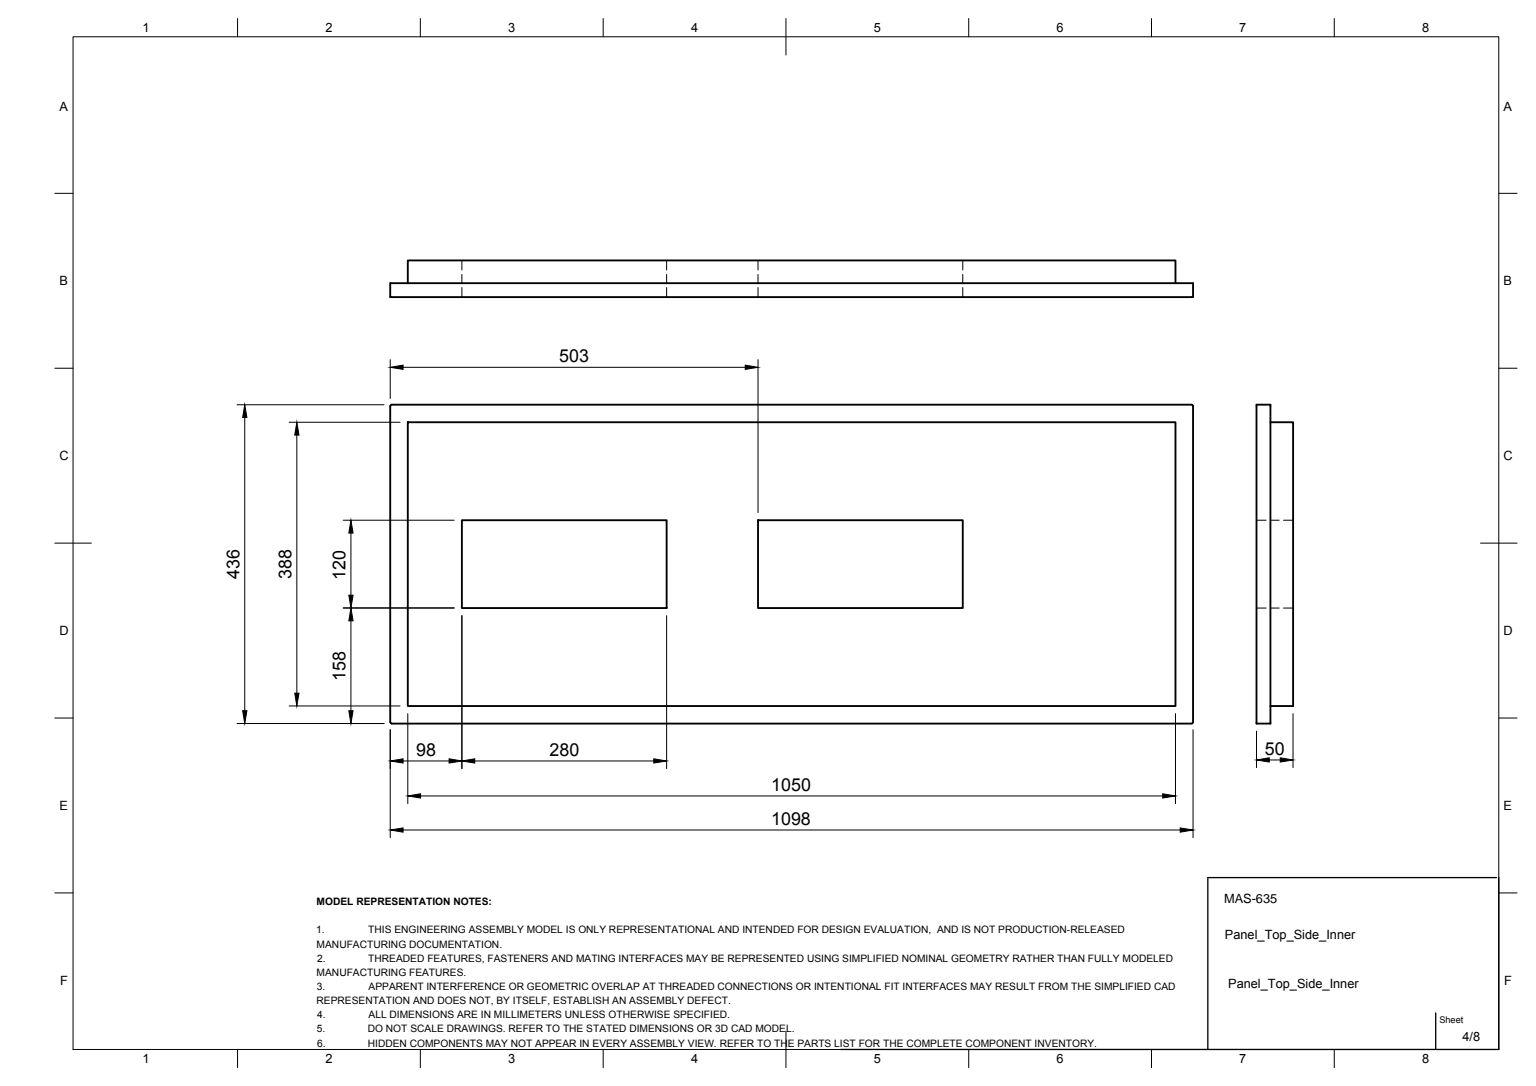
ISO-10303-21;
HEADER;
FILE_DESCRIPTION((''),'2;1');
FILE_NAME('Panel_Top_Side_Inner.step','2026-10-09T12:34:24-07:00',(''),(''),'','','');
FILE_SCHEMA (('AUTOMOTIVE_DESIGN { 1 0 10303 214 3 1 1 }'));
ENDSEC;
DATA;
#10=MECHANICAL_DESIGN_GEOMETRIC_PRESENTATION_REPRESENTATION('',(#60),#3759);
#48=SHAPE_REPRESENTATION_RELATIONSHIP('SRR','None',#3789,#54) ;
#54=ADVANCED_BREP_SHAPE_REPRESENTATION('',(#66),#3754) ;
#60=STYLED_ITEM('',(#3827),#66) ;
#66=MANIFOLD_SOLID_BREP('Body1',#2264) ;
#75=CYLINDRICAL_SURFACE('',#2389,0.2) ;
#76=CYLINDRICAL_SURFACE('',#2390,0.2) ;
#77=CYLINDRICAL_SURFACE('',#2391,0.2) ;
#78=CYLINDRICAL_SURFACE('',#2392,0.2) ;
#95=CIRCLE('',#2380,0.2) ;
#96=CIRCLE('',#2381,0.2) ;
#97=CIRCLE('',#2382,0.2) ;
#98=CIRCLE('',#2383,0.2) ;
#99=CIRCLE('',#2385,0.2) ;
#100=CIRCLE('',#2386,0.2) ;
#101=CIRCLE('',#2387,0.2) ;
#102=CIRCLE('',#2388,0.2) ;
#124=FACE_BOUND('',#294,.T.) ;
#125=FACE_BOUND('',#295,.T.) ;
#126=FACE_BOUND('',#301,.T.) ;
#127=FACE_BOUND('',#303,.T.) ;
#128=FACE_BOUND('',#304,.T.) ;
#164=FACE_OUTER_BOUND('',#289,.T.) ;
#165=FACE_OUTER_BOUND('',#290,.T.) ;
#166=FACE_OUTER_BOUND('',#291,.T.) ;
#167=FACE_OUTER_BOUND('',#292,.T.) ;
#168=FACE_OUTER_BOUND('',#293,.T.) ;
#169=FACE_OUTER_BOUND('',#296,.T.) ;
#170=FACE_OUTER_BOUND('',#297,.T.) ;
#171=FACE_OUTER_BOUND('',#298,.T.) ;
#172=FACE_OUTER_BOUND('',#299,.T.) ;
#173=FACE_OUTER_BOUND('',#300,.T.) ;
#174=FACE_OUTER_BOUND('',#302,.T.) ;
#175=FACE_OUTER_BOUND('',#305,.T.) ;
#176=FACE_OUTER_BOUND('',#306,.T.) ;
#177=FACE_OUTER_BOUND('',#307,.T.) ;
#178=FACE_OUTER_BOUND('',#308,.T.) ;
#179=FACE_OUTER_BOUND('',#309,.T.) ;
#180=FACE_OUTER_BOUND('',#310,.T.) ;
#181=FACE_OUTER_BOUND('',#311,.T.) ;
#182=FACE_OUTER_BOUND('',#312,.T.) ;
#183=FACE_OUTER_BOUND('',#313,.T.) ;
#184=FACE_OUTER_BOUND('',#314,.T.) ;
#185=FACE_OUTER_BOUND('',#315,.T.) ;
#186=FACE_OUTER_BOUND('',#316,.T.) ;
#289=EDGE_LOOP('',(#1559,#1560,#1561,#1562)) ;
#290=EDGE_LOOP('',(#1563,#1564,#1565,#1566)) ;
#291=EDGE_LOOP('',(#1567,#1568,#1569,#1570)) ;
#292=EDGE_LOOP('',(#1571,#1572,#1573,#1574)) ;
#293=EDGE_LOOP('',(#1575,#1576,#1577,#1578)) ;
#294=EDGE_LOOP('',(#1579,#1580,#1581,#1582)) ;
#295=EDGE_LOOP('',(#1583,#1584,#1585,#1586)) ;
#296=EDGE_LOOP('',(#1587,#1588,#1589,#1590)) ;
#297=EDGE_LOOP('',(#1591,#1592,#1593,#1594)) ;
#298=EDGE_LOOP('',(#1595,#1596,#1597,#1598)) ;
#299=EDGE_LOOP('',(#1599,#1600,#1601,#1602)) ;
#300=EDGE_LOOP('',(#1603,#1604,#1605,#1606,#1607,#1608,#1609,#1610)) ;
#301=EDGE_LOOP('',(#1611,#1612,#1613,#1614)) ;
#302=EDGE_LOOP('',(#1615,#1616,#1617,#1618,#1619,#1620,#1621,#1622)) ;
#303=EDGE_LOOP('',(#1623,#1624,#1625,#1626)) ;
#304=EDGE_LOOP('',(#1627,#1628,#1629,#1630)) ;
#305=EDGE_LOOP('',(#1631,#1632,#1633,#1634)) ;
#306=EDGE_LOOP('',(#1635,#1636,#1637,#1638)) ;
#307=EDGE_LOOP('',(#1639,#1640,#1641,#1642)) ;
#308=EDGE_LOOP('',(#1643,#1644,#1645,#1646)) ;
#309=EDGE_LOOP('',(#1647,#1648,#1649,#1650)) ;
#310=EDGE_LOOP('',(#1651,#1652,#1653,#1654)) ;
#311=EDGE_LOOP('',(#1655,#1656,#1657,#1658)) ;
#312=EDGE_LOOP('',(#1659,#1660,#1661,#1662)) ;
#313=EDGE_LOOP('',(#1663,#1664,#1665,#1666)) ;
#314=EDGE_LOOP('',(#1667,#1668,#1669,#1670)) ;
#315=EDGE_LOOP('',(#1671,#1672,#1673,#1674)) ;
#316=EDGE_LOOP('',(#1675,#1676,#1677,#1678)) ;
#455=LINE('',#3237,#723) ;
#456=LINE('',#3239,#724) ;
#457=LINE('',#3241,#725) ;
#458=LINE('',#3242,#726) ;
#459=LINE('',#3245,#727) ;
#460=LINE('',#3247,#728) ;
#461=LINE('',#3248,#729) ;
#462=LINE('',#3251,#730) ;
#463=LINE('',#3253,#731) ;
#464=LINE('',#3254,#732) ;
#465=LINE('',#3256,#733) ;
#466=LINE('',#3257,#734) ;
#467=LINE('',#3261,#735) ;
#468=LINE('',#3263,#736) ;
#469=LINE('',#3265,#737) ;
#470=LINE('',#3266,#738) ;
#471=LINE('',#3269,#739) ;
#472=LINE('',#3271,#740) ;
#473=LINE('',#3273,#741) ;
#474=LINE('',#3274,#742) ;
#475=LINE('',#3278,#743) ;
#476=LINE('',#3280,#744) ;
#477=LINE('',#3282,#745) ;
#478=LINE('',#3283,#746) ;
#479=LINE('',#3287,#747) ;
#480=LINE('',#3289,#748) ;
#481=LINE('',#3291,#749) ;
#482=LINE('',#3292,#750) ;
#483=LINE('',#3296,#751) ;
#484=LINE('',#3298,#752) ;
#485=LINE('',#3300,#753) ;
#486=LINE('',#3301,#754) ;
#487=LINE('',#3305,#755) ;
#488=LINE('',#3307,#756) ;
#489=LINE('',#3309,#757) ;
#490=LINE('',#3310,#758) ;
#491=LINE('',#3323,#759) ;
#492=LINE('',#3325,#760) ;
#493=LINE('',#3327,#761) ;
#494=LINE('',#3328,#762) ;
#495=LINE('',#3331,#763) ;
#496=LINE('',#3333,#764) ;
#497=LINE('',#3335,#765) ;
#498=LINE('',#3336,#766) ;
#499=LINE('',#3342,#767) ;
#500=LINE('',#3343,#768) ;
#501=LINE('',#3345,#769) ;
#502=LINE('',#3347,#770) ;
#503=LINE('',#3350,#771) ;
#504=LINE('',#3351,#772) ;
#505=LINE('',#3353,#773) ;
#506=LINE('',#3355,#774) ;
#723=VECTOR('',#2626,100.) ;
#724=VECTOR('',#2627,100.) ;
#725=VECTOR('',#2628,100.) ;
#726=VECTOR('',#2629,100.) ;
#727=VECTOR('',#2632,100.) ;
#728=VECTOR('',#2633,100.) ;
#729=VECTOR('',#2634,100.) ;
#730=VECTOR('',#2637,100.) ;
#731=VECTOR('',#2638,100.) ;
#732=VECTOR('',#2639,100.) ;
#733=VECTOR('',#2642,100.) ;
#734=VECTOR('',#2643,100.) ;
#735=VECTOR('',#2646,100.) ;
#736=VECTOR('',#2647,100.) ;
#737=VECTOR('',#2648,100.) ;
#738=VECTOR('',#2649,100.) ;
#739=VECTOR('',#2650,100.) ;
#740=VECTOR('',#2651,100.) ;
#741=VECTOR('',#2652,100.) ;
#742=VECTOR('',#2653,100.) ;
#743=VECTOR('',#2656,100.) ;
#744=VECTOR('',#2657,100.) ;
#745=VECTOR('',#2658,100.) ;
#746=VECTOR('',#2659,100.) ;
#747=VECTOR('',#2662,100.) ;
#748=VECTOR('',#2663,100.) ;
#749=VECTOR('',#2664,100.) ;
#750=VECTOR('',#2665,100.) ;
#751=VECTOR('',#2668,100.) ;
#752=VECTOR('',#2669,100.) ;
#753=VECTOR('',#2670,100.) ;
#754=VECTOR('',#2671,100.) ;
#755=VECTOR('',#2674,100.) ;
#756=VECTOR('',#2675,100.) ;
#757=VECTOR('',#2676,100.) ;
#758=VECTOR('',#2677,100.) ;
#759=VECTOR('',#2698,100.) ;
#760=VECTOR('',#2699,100.) ;
#761=VECTOR('',#2700,100.) ;
#762=VECTOR('',#2701,100.) ;
#763=VECTOR('',#2702,100.) ;
#764=VECTOR('',#2703,100.) ;
#765=VECTOR('',#2704,100.) ;
#766=VECTOR('',#2705,100.) ;
#767=VECTOR('',#2716,100.) ;
#768=VECTOR('',#2717,100.) ;
#769=VECTOR('',#2720,100.) ;
#770=VECTOR('',#2723,100.) ;
#771=VECTOR('',#2728,100.) ;
#772=VECTOR('',#2729,100.) ;
#773=VECTOR('',#2732,100.) ;
#774=VECTOR('',#2735,100.) ;
#979=VERTEX_POINT('',#3235) ;
#980=VERTEX_POINT('',#3236) ;
#981=VERTEX_POINT('',#3238) ;
#982=VERTEX_POINT('',#3240) ;
#983=VERTEX_POINT('',#3244) ;
#984=VERTEX_POINT('',#3246) ;
#985=VERTEX_POINT('',#3250) ;
#986=VERTEX_POINT('',#3252) ;
#987=VERTEX_POINT('',#3259) ;
#988=VERTEX_POINT('',#3260) ;
#989=VERTEX_POINT('',#3262) ;
#990=VERTEX_POINT('',#3264) ;
#991=VERTEX_POINT('',#3267) ;
#992=VERTEX_POINT('',#3268) ;
#993=VERTEX_POINT('',#3270) ;
#994=VERTEX_POINT('',#3272) ;
#995=VERTEX_POINT('',#3276) ;
#996=VERTEX_POINT('',#3277) ;
#997=VERTEX_POINT('',#3279) ;
#998=VERTEX_POINT('',#3281) ;
#999=VERTEX_POINT('',#3285) ;
#1000=VERTEX_POINT('',#3286) ;
#1001=VERTEX_POINT('',#3288) ;
#1002=VERTEX_POINT('',#3290) ;
#1003=VERTEX_POINT('',#3294) ;
#1004=VERTEX_POINT('',#3295) ;
#1005=VERTEX_POINT('',#3297) ;
#1006=VERTEX_POINT('',#3299) ;
#1007=VERTEX_POINT('',#3303) ;
#1008=VERTEX_POINT('',#3304) ;
#1009=VERTEX_POINT('',#3306) ;
#1010=VERTEX_POINT('',#3308) ;
#1011=VERTEX_POINT('',#3321) ;
#1012=VERTEX_POINT('',#3322) ;
#1013=VERTEX_POINT('',#3324) ;
#1014=VERTEX_POINT('',#3326) ;
#1015=VERTEX_POINT('',#3329) ;
#1016=VERTEX_POINT('',#3330) ;
#1017=VERTEX_POINT('',#3332) ;
#1018=VERTEX_POINT('',#3334) ;
#1199=EDGE_CURVE('',#979,#980,#455,.T.) ;
#1200=EDGE_CURVE('',#981,#979,#456,.T.) ;
#1201=EDGE_CURVE('',#981,#982,#457,.T.) ;
#1202=EDGE_CURVE('',#982,#980,#458,.T.) ;
#1203=EDGE_CURVE('',#979,#983,#459,.T.) ;
#1204=EDGE_CURVE('',#984,#983,#460,.T.) ;
#1205=EDGE_CURVE('',#981,#984,#461,.T.) ;
#1206=EDGE_CURVE('',#983,#985,#462,.T.) ;
#1207=EDGE_CURVE('',#986,#985,#463,.T.) ;
#1208=EDGE_CURVE('',#984,#986,#464,.T.) ;
#1209=EDGE_CURVE('',#980,#985,#465,.T.) ;
#1210=EDGE_CURVE('',#982,#986,#466,.T.) ;
#1211=EDGE_CURVE('',#987,#988,#467,.T.) ;
#1212=EDGE_CURVE('',#988,#989,#468,.T.) ;
#1213=EDGE_CURVE('',#989,#990,#469,.T.) ;
#1214=EDGE_CURVE('',#990,#987,#470,.T.) ;
#1215=EDGE_CURVE('',#991,#992,#471,.T.) ;
#1216=EDGE_CURVE('',#992,#993,#472,.T.) ;
#1217=EDGE_CURVE('',#993,#994,#473,.T.) ;
#1218=EDGE_CURVE('',#994,#991,#474,.T.) ;
#1219=EDGE_CURVE('',#995,#996,#475,.T.) ;
#1220=EDGE_CURVE('',#995,#997,#476,.T.) ;
#1221=EDGE_CURVE('',#997,#998,#477,.T.) ;
#1222=EDGE_CURVE('',#998,#996,#478,.T.) ;
#1223=EDGE_CURVE('',#999,#1000,#479,.T.) ;
#1224=EDGE_CURVE('',#1000,#1001,#480,.T.) ;
#1225=EDGE_CURVE('',#1002,#1001,#481,.T.) ;
#1226=EDGE_CURVE('',#1002,#999,#482,.T.) ;
#1227=EDGE_CURVE('',#1003,#1004,#483,.T.) ;
#1228=EDGE_CURVE('',#1003,#1005,#484,.T.) ;
#1229=EDGE_CURVE('',#1005,#1006,#485,.T.) ;
#1230=EDGE_CURVE('',#1006,#1004,#486,.T.) ;
#1231=EDGE_CURVE('',#1007,#1008,#487,.T.) ;
#1232=EDGE_CURVE('',#1007,#1009,#488,.T.) ;
#1233=EDGE_CURVE('',#1009,#1010,#489,.T.) ;
#1234=EDGE_CURVE('',#1010,#1008,#490,.T.) ;
#1235=EDGE_CURVE('',#1009,#995,#95,.T.) ;
#1236=EDGE_CURVE('',#996,#1002,#96,.T.) ;
#1237=EDGE_CURVE('',#1001,#1006,#97,.T.) ;
#1238=EDGE_CURVE('',#1005,#1010,#98,.T.) ;
#1239=EDGE_CURVE('',#997,#1007,#99,.T.) ;
#1240=EDGE_CURVE('',#1008,#1003,#100,.T.) ;
#1241=EDGE_CURVE('',#1004,#1000,#101,.T.) ;
#1242=EDGE_CURVE('',#999,#998,#102,.T.) ;
#1243=EDGE_CURVE('',#1011,#1012,#491,.T.) ;
#1244=EDGE_CURVE('',#1013,#1011,#492,.T.) ;
#1245=EDGE_CURVE('',#1014,#1013,#493,.T.) ;
#1246=EDGE_CURVE('',#1012,#1014,#494,.T.) ;
#1247=EDGE_CURVE('',#1015,#1016,#495,.T.) ;
#1248=EDGE_CURVE('',#1017,#1015,#496,.T.) ;
#1249=EDGE_CURVE('',#1018,#1017,#497,.T.) ;
#1250=EDGE_CURVE('',#1016,#1018,#498,.T.) ;
#1251=EDGE_CURVE('',#992,#1015,#499,.T.) ;
#1252=EDGE_CURVE('',#993,#1016,#500,.T.) ;
#1253=EDGE_CURVE('',#991,#1017,#501,.T.) ;
#1254=EDGE_CURVE('',#994,#1018,#502,.T.) ;
#1255=EDGE_CURVE('',#988,#1011,#503,.T.) ;
#1256=EDGE_CURVE('',#989,#1012,#504,.T.) ;
#1257=EDGE_CURVE('',#987,#1013,#505,.T.) ;
#1258=EDGE_CURVE('',#990,#1014,#506,.T.) ;
#1559=ORIENTED_EDGE('',*,*,#1199,.F.) ;
#1560=ORIENTED_EDGE('',*,*,#1200,.F.) ;
#1561=ORIENTED_EDGE('',*,*,#1201,.T.) ;
#1562=ORIENTED_EDGE('',*,*,#1202,.T.) ;
#1563=ORIENTED_EDGE('',*,*,#1200,.T.) ;
#1564=ORIENTED_EDGE('',*,*,#1203,.T.) ;
#1565=ORIENTED_EDGE('',*,*,#1204,.F.) ;
#1566=ORIENTED_EDGE('',*,*,#1205,.F.) ;
#1567=ORIENTED_EDGE('',*,*,#1204,.T.) ;
#1568=ORIENTED_EDGE('',*,*,#1206,.T.) ;
#1569=ORIENTED_EDGE('',*,*,#1207,.F.) ;
#1570=ORIENTED_EDGE('',*,*,#1208,.F.) ;
#1571=ORIENTED_EDGE('',*,*,#1209,.F.) ;
#1572=ORIENTED_EDGE('',*,*,#1202,.F.) ;
#1573=ORIENTED_EDGE('',*,*,#1210,.T.) ;
#1574=ORIENTED_EDGE('',*,*,#1207,.T.) ;
#1575=ORIENTED_EDGE('',*,*,#1201,.F.) ;
#1576=ORIENTED_EDGE('',*,*,#1205,.T.) ;
#1577=ORIENTED_EDGE('',*,*,#1208,.T.) ;
#1578=ORIENTED_EDGE('',*,*,#1210,.F.) ;
#1579=ORIENTED_EDGE('',*,*,#1211,.T.) ;
#1580=ORIENTED_EDGE('',*,*,#1212,.T.) ;
#1581=ORIENTED_EDGE('',*,*,#1213,.T.) ;
#1582=ORIENTED_EDGE('',*,*,#1214,.T.) ;
#1583=ORIENTED_EDGE('',*,*,#1215,.T.) ;
#1584=ORIENTED_EDGE('',*,*,#1216,.T.) ;
#1585=ORIENTED_EDGE('',*,*,#1217,.T.) ;
#1586=ORIENTED_EDGE('',*,*,#1218,.T.) ;
#1587=ORIENTED_EDGE('',*,*,#1219,.F.) ;
#1588=ORIENTED_EDGE('',*,*,#1220,.T.) ;
#1589=ORIENTED_EDGE('',*,*,#1221,.T.) ;
#1590=ORIENTED_EDGE('',*,*,#1222,.T.) ;
#1591=ORIENTED_EDGE('',*,*,#1223,.T.) ;
#1592=ORIENTED_EDGE('',*,*,#1224,.T.) ;
#1593=ORIENTED_EDGE('',*,*,#1225,.F.) ;
#1594=ORIENTED_EDGE('',*,*,#1226,.T.) ;
#1595=ORIENTED_EDGE('',*,*,#1227,.F.) ;
#1596=ORIENTED_EDGE('',*,*,#1228,.T.) ;
#1597=ORIENTED_EDGE('',*,*,#1229,.T.) ;
#1598=ORIENTED_EDGE('',*,*,#1230,.T.) ;
#1599=ORIENTED_EDGE('',*,*,#1231,.F.) ;
#1600=ORIENTED_EDGE('',*,*,#1232,.T.) ;
#1601=ORIENTED_EDGE('',*,*,#1233,.T.) ;
#1602=ORIENTED_EDGE('',*,*,#1234,.T.) ;
#1603=ORIENTED_EDGE('',*,*,#1233,.F.) ;
#1604=ORIENTED_EDGE('',*,*,#1235,.T.) ;
#1605=ORIENTED_EDGE('',*,*,#1219,.T.) ;
#1606=ORIENTED_EDGE('',*,*,#1236,.T.) ;
#1607=ORIENTED_EDGE('',*,*,#1225,.T.) ;
#1608=ORIENTED_EDGE('',*,*,#1237,.T.) ;
#1609=ORIENTED_EDGE('',*,*,#1229,.F.) ;
#1610=ORIENTED_EDGE('',*,*,#1238,.T.) ;
#1611=ORIENTED_EDGE('',*,*,#1203,.F.) ;
#1612=ORIENTED_EDGE('',*,*,#1199,.T.) ;
#1613=ORIENTED_EDGE('',*,*,#1209,.T.) ;
#1614=ORIENTED_EDGE('',*,*,#1206,.F.) ;
#1615=ORIENTED_EDGE('',*,*,#1221,.F.) ;
#1616=ORIENTED_EDGE('',*,*,#1239,.T.) ;
#1617=ORIENTED_EDGE('',*,*,#1231,.T.) ;
#1618=ORIENTED_EDGE('',*,*,#1240,.T.) ;
#1619=ORIENTED_EDGE('',*,*,#1227,.T.) ;
#1620=ORIENTED_EDGE('',*,*,#1241,.T.) ;
#1621=ORIENTED_EDGE('',*,*,#1223,.F.) ;
#1622=ORIENTED_EDGE('',*,*,#1242,.T.) ;
#1623=ORIENTED_EDGE('',*,*,#1243,.F.) ;
#1624=ORIENTED_EDGE('',*,*,#1244,.F.) ;
#1625=ORIENTED_EDGE('',*,*,#1245,.F.) ;
#1626=ORIENTED_EDGE('',*,*,#1246,.F.) ;
#1627=ORIENTED_EDGE('',*,*,#1247,.F.) ;
#1628=ORIENTED_EDGE('',*,*,#1248,.F.) ;
#1629=ORIENTED_EDGE('',*,*,#1249,.F.) ;
#1630=ORIENTED_EDGE('',*,*,#1250,.F.) ;
#1631=ORIENTED_EDGE('',*,*,#1235,.F.) ;
#1632=ORIENTED_EDGE('',*,*,#1232,.F.) ;
#1633=ORIENTED_EDGE('',*,*,#1239,.F.) ;
#1634=ORIENTED_EDGE('',*,*,#1220,.F.) ;
#1635=ORIENTED_EDGE('',*,*,#1238,.F.) ;
#1636=ORIENTED_EDGE('',*,*,#1228,.F.) ;
#1637=ORIENTED_EDGE('',*,*,#1240,.F.) ;
#1638=ORIENTED_EDGE('',*,*,#1234,.F.) ;
#1639=ORIENTED_EDGE('',*,*,#1237,.F.) ;
#1640=ORIENTED_EDGE('',*,*,#1224,.F.) ;
#1641=ORIENTED_EDGE('',*,*,#1241,.F.) ;
#1642=ORIENTED_EDGE('',*,*,#1230,.F.) ;
#1643=ORIENTED_EDGE('',*,*,#1236,.F.) ;
#1644=ORIENTED_EDGE('',*,*,#1222,.F.) ;
#1645=ORIENTED_EDGE('',*,*,#1242,.F.) ;
#1646=ORIENTED_EDGE('',*,*,#1226,.F.) ;
#1647=ORIENTED_EDGE('',*,*,#1251,.T.) ;
#1648=ORIENTED_EDGE('',*,*,#1247,.T.) ;
#1649=ORIENTED_EDGE('',*,*,#1252,.F.) ;
#1650=ORIENTED_EDGE('',*,*,#1216,.F.) ;
#1651=ORIENTED_EDGE('',*,*,#1253,.T.) ;
#1652=ORIENTED_EDGE('',*,*,#1248,.T.) ;
#1653=ORIENTED_EDGE('',*,*,#1251,.F.) ;
#1654=ORIENTED_EDGE('',*,*,#1215,.F.) ;
#1655=ORIENTED_EDGE('',*,*,#1254,.T.) ;
#1656=ORIENTED_EDGE('',*,*,#1249,.T.) ;
#1657=ORIENTED_EDGE('',*,*,#1253,.F.) ;
#1658=ORIENTED_EDGE('',*,*,#1218,.F.) ;
#1659=ORIENTED_EDGE('',*,*,#1252,.T.) ;
#1660=ORIENTED_EDGE('',*,*,#1250,.T.) ;
#1661=ORIENTED_EDGE('',*,*,#1254,.F.) ;
#1662=ORIENTED_EDGE('',*,*,#1217,.F.) ;
#1663=ORIENTED_EDGE('',*,*,#1255,.T.) ;
#1664=ORIENTED_EDGE('',*,*,#1243,.T.) ;
#1665=ORIENTED_EDGE('',*,*,#1256,.F.) ;
#1666=ORIENTED_EDGE('',*,*,#1212,.F.) ;
#1667=ORIENTED_EDGE('',*,*,#1257,.T.) ;
#1668=ORIENTED_EDGE('',*,*,#1244,.T.) ;
#1669=ORIENTED_EDGE('',*,*,#1255,.F.) ;
#1670=ORIENTED_EDGE('',*,*,#1211,.F.) ;
#1671=ORIENTED_EDGE('',*,*,#1258,.T.) ;
#1672=ORIENTED_EDGE('',*,*,#1245,.T.) ;
#1673=ORIENTED_EDGE('',*,*,#1257,.F.) ;
#1674=ORIENTED_EDGE('',*,*,#1214,.F.) ;
#1675=ORIENTED_EDGE('',*,*,#1256,.T.) ;
#1676=ORIENTED_EDGE('',*,*,#1246,.T.) ;
#1677=ORIENTED_EDGE('',*,*,#1258,.F.) ;
#1678=ORIENTED_EDGE('',*,*,#1213,.F.) ;
#2058=PLANE('',#2370) ;
#2059=PLANE('',#2371) ;
#2060=PLANE('',#2372) ;
#2061=PLANE('',#2373) ;
#2062=PLANE('',#2374) ;
#2063=PLANE('',#2375) ;
#2064=PLANE('',#2376) ;
#2065=PLANE('',#2377) ;
#2066=PLANE('',#2378) ;
#2067=PLANE('',#2379) ;
#2068=PLANE('',#2384) ;
#2069=PLANE('',#2393) ;
#2070=PLANE('',#2394) ;
#2071=PLANE('',#2395) ;
#2072=PLANE('',#2396) ;
#2073=PLANE('',#2397) ;
#2074=PLANE('',#2398) ;
#2075=PLANE('',#2399) ;
#2076=PLANE('',#2400) ;
#2166=ADVANCED_FACE('',(#164),#2058,.T.) ;
#2167=ADVANCED_FACE('',(#165),#2059,.F.) ;
#2168=ADVANCED_FACE('',(#166),#2060,.F.) ;
#2169=ADVANCED_FACE('',(#167),#2061,.T.) ;
#2170=ADVANCED_FACE('',(#168,#124,#125),#2062,.F.) ;
#2171=ADVANCED_FACE('',(#169),#2063,.F.) ;
#2172=ADVANCED_FACE('',(#170),#2064,.F.) ;
#2173=ADVANCED_FACE('',(#171),#2065,.T.) ;
#2174=ADVANCED_FACE('',(#172),#2066,.T.) ;
#2175=ADVANCED_FACE('',(#173,#126),#2067,.T.) ;
#2176=ADVANCED_FACE('',(#174,#127,#128),#2068,.T.) ;
#2177=ADVANCED_FACE('',(#175),#75,.T.) ;
#2178=ADVANCED_FACE('',(#176),#76,.T.) ;
#2179=ADVANCED_FACE('',(#177),#77,.T.) ;
#2180=ADVANCED_FACE('',(#178),#78,.T.) ;
#2181=ADVANCED_FACE('',(#179),#2069,.F.) ;
#2182=ADVANCED_FACE('',(#180),#2070,.F.) ;
#2183=ADVANCED_FACE('',(#181),#2071,.F.) ;
#2184=ADVANCED_FACE('',(#182),#2072,.F.) ;
#2185=ADVANCED_FACE('',(#183),#2073,.F.) ;
#2186=ADVANCED_FACE('',(#184),#2074,.F.) ;
#2187=ADVANCED_FACE('',(#185),#2075,.F.) ;
#2188=ADVANCED_FACE('',(#186),#2076,.F.) ;
#2264=CLOSED_SHELL('',(#2166,#2167,#2168,#2169,#2170,#2171,#2172,#2173,
#2174,#2175,#2176,#2177,#2178,#2179,#2180,#2181,#2182,#2183,#2184,#2185,
#2186,#2187,#2188)) ;
#2369=AXIS2_PLACEMENT_3D('',#3233,#2622,#2623) ;
#2370=AXIS2_PLACEMENT_3D('',#3234,#2624,#2625) ;
#2371=AXIS2_PLACEMENT_3D('',#3243,#2630,#2631) ;
#2372=AXIS2_PLACEMENT_3D('',#3249,#2635,#2636) ;
#2373=AXIS2_PLACEMENT_3D('',#3255,#2640,#2641) ;
#2374=AXIS2_PLACEMENT_3D('',#3258,#2644,#2645) ;
#2375=AXIS2_PLACEMENT_3D('',#3275,#2654,#2655) ;
#2376=AXIS2_PLACEMENT_3D('',#3284,#2660,#2661) ;
#2377=AXIS2_PLACEMENT_3D('',#3293,#2666,#2667) ;
#2378=AXIS2_PLACEMENT_3D('',#3302,#2672,#2673) ;
#2379=AXIS2_PLACEMENT_3D('',#3311,#2678,#2679) ;
#2380=AXIS2_PLACEMENT_3D('',#3312,#2680,#2681) ;
#2381=AXIS2_PLACEMENT_3D('',#3313,#2682,#2683) ;
#2382=AXIS2_PLACEMENT_3D('',#3314,#2684,#2685) ;
#2383=AXIS2_PLACEMENT_3D('',#3315,#2686,#2687) ;
#2384=AXIS2_PLACEMENT_3D('',#3316,#2688,#2689) ;
#2385=AXIS2_PLACEMENT_3D('',#3317,#2690,#2691) ;
#2386=AXIS2_PLACEMENT_3D('',#3318,#2692,#2693) ;
#2387=AXIS2_PLACEMENT_3D('',#3319,#2694,#2695) ;
#2388=AXIS2_PLACEMENT_3D('',#3320,#2696,#2697) ;
#2389=AXIS2_PLACEMENT_3D('',#3337,#2706,#2707) ;
#2390=AXIS2_PLACEMENT_3D('',#3338,#2708,#2709) ;
#2391=AXIS2_PLACEMENT_3D('',#3339,#2710,#2711) ;
#2392=AXIS2_PLACEMENT_3D('',#3340,#2712,#2713) ;
#2393=AXIS2_PLACEMENT_3D('',#3341,#2714,#2715) ;
#2394=AXIS2_PLACEMENT_3D('',#3344,#2718,#2719) ;
#2395=AXIS2_PLACEMENT_3D('',#3346,#2721,#2722) ;
#2396=AXIS2_PLACEMENT_3D('',#3348,#2724,#2725) ;
#2397=AXIS2_PLACEMENT_3D('',#3349,#2726,#2727) ;
#2398=AXIS2_PLACEMENT_3D('',#3352,#2730,#2731) ;
#2399=AXIS2_PLACEMENT_3D('',#3354,#2733,#2734) ;
#2400=AXIS2_PLACEMENT_3D('',#3356,#2736,#2737) ;
#2622=DIRECTION('axis',(0.,0.,1.)) ;
#2623=DIRECTION('refdir',(1.,0.,0.)) ;
#2624=DIRECTION('center_axis',(1.58603289232165E-16,-1.,0.)) ;
#2625=DIRECTION('ref_axis',(1.,1.58603289232165E-16,0.)) ;
#2626=DIRECTION('',(-1.,-1.58603289232165E-16,0.)) ;
#2627=DIRECTION('',(0.,0.,-1.)) ;
#2628=DIRECTION('',(-1.,-1.58603289232165E-16,0.)) ;
#2629=DIRECTION('',(0.,0.,-1.)) ;
#2630=DIRECTION('center_axis',(-1.,0.,0.)) ;
#2631=DIRECTION('ref_axis',(0.,0.,1.)) ;
#2632=DIRECTION('',(0.,1.,0.)) ;
#2633=DIRECTION('',(0.,0.,-1.)) ;
#2634=DIRECTION('',(0.,1.,0.)) ;
#2635=DIRECTION('center_axis',(1.05735526154777E-16,-1.,0.)) ;
#2636=DIRECTION('ref_axis',(1.,1.05735526154777E-16,0.)) ;
#2637=DIRECTION('',(-1.,-1.05735526154777E-16,0.)) ;
#2638=DIRECTION('',(0.,0.,-1.)) ;
#2639=DIRECTION('',(-1.,-1.05735526154777E-16,0.)) ;
#2640=DIRECTION('center_axis',(-1.,0.,0.)) ;
#2641=DIRECTION('ref_axis',(0.,0.,1.)) ;
#2642=DIRECTION('',(0.,1.,0.)) ;
#2643=DIRECTION('',(0.,1.,0.)) ;
#2644=DIRECTION('center_axis',(0.,0.,-1.)) ;
#2645=DIRECTION('ref_axis',(-1.,0.,0.)) ;
#2646=DIRECTION('',(1.,-1.23908819712629E-16,0.)) ;
#2647=DIRECTION('',(0.,-1.,0.)) ;
#2648=DIRECTION('',(-1.,1.23908819712629E-16,0.)) ;
#2649=DIRECTION('',(0.,1.,0.)) ;
#2650=DIRECTION('',(-1.,0.,0.)) ;
#2651=DIRECTION('',(0.,1.,0.)) ;
#2652=DIRECTION('',(1.,0.,0.)) ;
#2653=DIRECTION('',(0.,-1.,0.)) ;
#2654=DIRECTION('center_axis',(-1.,0.,0.)) ;
#2655=DIRECTION('ref_axis',(0.,0.,1.)) ;
#2656=DIRECTION('',(0.,1.,0.)) ;
#2657=DIRECTION('',(0.,0.,-1.)) ;
#2658=DIRECTION('',(0.,1.,0.)) ;
#2659=DIRECTION('',(0.,0.,1.)) ;
#2660=DIRECTION('center_axis',(1.26391510089385E-16,-1.,0.)) ;
#2661=DIRECTION('ref_axis',(1.,1.26391510089385E-16,0.)) ;
#2662=DIRECTION('',(-1.,-1.26391510089385E-16,0.)) ;
#2663=DIRECTION('',(0.,0.,1.)) ;
#2664=DIRECTION('',(-1.,-1.26391510089385E-16,0.)) ;
#2665=DIRECTION('',(0.,0.,-1.)) ;
#2666=DIRECTION('center_axis',(-1.,0.,0.)) ;
#2667=DIRECTION('ref_axis',(0.,0.,1.)) ;
#2668=DIRECTION('',(0.,1.,0.)) ;
#2669=DIRECTION('',(0.,0.,1.)) ;
#2670=DIRECTION('',(0.,1.,0.)) ;
#2671=DIRECTION('',(0.,0.,-1.)) ;
#2672=DIRECTION('center_axis',(1.51669812107262E-16,-1.,0.)) ;
#2673=DIRECTION('ref_axis',(1.,1.51669812107262E-16,0.)) ;
#2674=DIRECTION('',(-1.,-1.51669812107262E-16,0.)) ;
#2675=DIRECTION('',(0.,0.,1.)) ;
#2676=DIRECTION('',(-1.,-1.51669812107262E-16,0.)) ;
#2677=DIRECTION('',(0.,0.,-1.)) ;
#2678=DIRECTION('center_axis',(0.,0.,1.)) ;
#2679=DIRECTION('ref_axis',(1.,0.,0.)) ;
#2680=DIRECTION('center_axis',(0.,0.,1.)) ;
#2681=DIRECTION('ref_axis',(1.,0.,0.)) ;
#2682=DIRECTION('center_axis',(0.,0.,1.)) ;
#2683=DIRECTION('ref_axis',(1.,0.,0.)) ;
#2684=DIRECTION('center_axis',(0.,0.,1.)) ;
#2685=DIRECTION('ref_axis',(1.,0.,0.)) ;
#2686=DIRECTION('center_axis',(0.,0.,1.)) ;
#2687=DIRECTION('ref_axis',(1.,0.,0.)) ;
#2688=DIRECTION('center_axis',(0.,0.,-1.)) ;
#2689=DIRECTION('ref_axis',(-1.,0.,0.)) ;
#2690=DIRECTION('center_axis',(0.,0.,-1.)) ;
#2691=DIRECTION('ref_axis',(-1.,0.,0.)) ;
#2692=DIRECTION('center_axis',(0.,0.,-1.)) ;
#2693=DIRECTION('ref_axis',(-1.,0.,0.)) ;
#2694=DIRECTION('center_axis',(0.,0.,-1.)) ;
#2695=DIRECTION('ref_axis',(-1.,0.,0.)) ;
#2696=DIRECTION('center_axis',(0.,0.,-1.)) ;
#2697=DIRECTION('ref_axis',(-1.,0.,0.)) ;
#2698=DIRECTION('',(0.,-1.,0.)) ;
#2699=DIRECTION('',(1.,-1.23908819712629E-16,0.)) ;
#2700=DIRECTION('',(0.,1.,0.)) ;
#2701=DIRECTION('',(-1.,1.23908819712629E-16,0.)) ;
#2702=DIRECTION('',(0.,1.,0.)) ;
#2703=DIRECTION('',(-1.,0.,0.)) ;
#2704=DIRECTION('',(0.,-1.,0.)) ;
#2705=DIRECTION('',(1.,0.,0.)) ;
#2706=DIRECTION('center_axis',(0.,0.,1.)) ;
#2707=DIRECTION('ref_axis',(1.,0.,0.)) ;
#2708=DIRECTION('center_axis',(0.,0.,-1.)) ;
#2709=DIRECTION('ref_axis',(-1.,0.,0.)) ;
#2710=DIRECTION('center_axis',(0.,0.,1.)) ;
#2711=DIRECTION('ref_axis',(1.,0.,0.)) ;
#2712=DIRECTION('center_axis',(0.,0.,-1.)) ;
#2713=DIRECTION('ref_axis',(-1.,0.,0.)) ;
#2714=DIRECTION('center_axis',(-1.,0.,0.)) ;
#2715=DIRECTION('ref_axis',(0.,0.,1.)) ;
#2716=DIRECTION('',(0.,0.,-1.)) ;
#2717=DIRECTION('',(0.,0.,-1.)) ;
#2718=DIRECTION('center_axis',(0.,-1.,0.)) ;
#2719=DIRECTION('ref_axis',(0.,0.,-1.)) ;
#2720=DIRECTION('',(0.,0.,-1.)) ;
#2721=DIRECTION('center_axis',(1.,0.,0.)) ;
#2722=DIRECTION('ref_axis',(0.,0.,-1.)) ;
#2723=DIRECTION('',(0.,0.,-1.)) ;
#2724=DIRECTION('center_axis',(0.,1.,0.)) ;
#2725=DIRECTION('ref_axis',(0.,0.,1.)) ;
#2726=DIRECTION('center_axis',(1.,0.,0.)) ;
#2727=DIRECTION('ref_axis',(0.,0.,-1.)) ;
#2728=DIRECTION('',(0.,0.,-1.)) ;
#2729=DIRECTION('',(0.,0.,-1.)) ;
#2730=DIRECTION('center_axis',(1.23908819712629E-16,1.,0.)) ;
#2731=DIRECTION('ref_axis',(-1.,1.23908819712629E-16,0.)) ;
#2732=DIRECTION('',(0.,0.,-1.)) ;
#2733=DIRECTION('center_axis',(-1.,0.,0.)) ;
#2734=DIRECTION('ref_axis',(0.,0.,1.)) ;
#2735=DIRECTION('',(0.,0.,-1.)) ;
#2736=DIRECTION('center_axis',(-1.23908819712629E-16,-1.,0.)) ;
#2737=DIRECTION('ref_axis',(1.,-1.23908819712629E-16,0.)) ;
#3233=CARTESIAN_POINT('',(0.,0.,0.)) ;
#3234=CARTESIAN_POINT('Origin',(52.5,-19.4,5.)) ;
#3235=CARTESIAN_POINT('',(52.5,-19.4,1.9)) ;
#3236=CARTESIAN_POINT('',(-52.5,-19.4,1.9)) ;
#3237=CARTESIAN_POINT('',(52.5,-19.4,1.9)) ;
#3238=CARTESIAN_POINT('',(52.5,-19.4,5.)) ;
#3239=CARTESIAN_POINT('',(52.5,-19.4,5.)) ;
#3240=CARTESIAN_POINT('',(-52.5,-19.4,5.)) ;
#3241=CARTESIAN_POINT('',(52.5,-19.4,5.)) ;
#3242=CARTESIAN_POINT('',(-52.5,-19.4,5.)) ;
#3243=CARTESIAN_POINT('Origin',(52.5,-19.4,5.)) ;
#3244=CARTESIAN_POINT('',(52.5,19.4,1.9)) ;
#3245=CARTESIAN_POINT('',(52.5,-19.4,1.9)) ;
#3246=CARTESIAN_POINT('',(52.5,19.4,5.)) ;
#3247=CARTESIAN_POINT('',(52.5,19.4,5.)) ;
#3248=CARTESIAN_POINT('',(52.5,-19.4,5.)) ;
#3249=CARTESIAN_POINT('Origin',(52.5,19.4,5.)) ;
#3250=CARTESIAN_POINT('',(-52.5,19.4,1.9)) ;
#3251=CARTESIAN_POINT('',(52.5,19.4,1.9)) ;
#3252=CARTESIAN_POINT('',(-52.5,19.4,5.)) ;
#3253=CARTESIAN_POINT('',(-52.5,19.4,5.)) ;
#3254=CARTESIAN_POINT('',(52.5,19.4,5.)) ;
#3255=CARTESIAN_POINT('Origin',(-52.5,-19.4,5.)) ;
#3256=CARTESIAN_POINT('',(-52.5,-19.4,1.9)) ;
#3257=CARTESIAN_POINT('',(-52.5,-19.4,5.)) ;
#3258=CARTESIAN_POINT('Origin',(0.,0.,5.)) ;
#3259=CARTESIAN_POINT('',(-4.6,6.00000000000001,5.)) ;
#3260=CARTESIAN_POINT('',(23.4,6.00000000000001,5.)) ;
#3261=CARTESIAN_POINT('',(7.43452918275775E-16,6.00000000000001,5.)) ;
#3262=CARTESIAN_POINT('',(23.4,-6.,5.)) ;
#3263=CARTESIAN_POINT('',(23.4,0.,5.)) ;
#3264=CARTESIAN_POINT('',(-4.6,-5.99999999999999,5.)) ;
#3265=CARTESIAN_POINT('',(-7.43452918275773E-16,-5.99999999999999,5.)) ;
#3266=CARTESIAN_POINT('',(-4.6,0.,5.)) ;
#3267=CARTESIAN_POINT('',(-17.1,-5.99999999999999,5.)) ;
#3268=CARTESIAN_POINT('',(-45.1,-5.99999999999999,5.)) ;
#3269=CARTESIAN_POINT('',(0.,-5.99999999999999,5.)) ;
#3270=CARTESIAN_POINT('',(-45.1,6.00000000000001,5.)) ;
#3271=CARTESIAN_POINT('',(-45.1,0.,5.)) ;
#3272=CARTESIAN_POINT('',(-17.1,6.00000000000001,5.)) ;
#3273=CARTESIAN_POINT('',(0.,6.00000000000001,5.)) ;
#3274=CARTESIAN_POINT('',(-17.1,0.,5.)) ;
#3275=CARTESIAN_POINT('Origin',(54.9,-21.8,1.9)) ;
#3276=CARTESIAN_POINT('',(54.9,-21.6,1.9)) ;
#3277=CARTESIAN_POINT('',(54.9,21.6,1.9)) ;
#3278=CARTESIAN_POINT('',(54.9,-21.8,1.9)) ;
#3279=CARTESIAN_POINT('',(54.9,-21.6,0.)) ;
#3280=CARTESIAN_POINT('',(54.9,-21.6,0.)) ;
#3281=CARTESIAN_POINT('',(54.9,21.6,0.)) ;
#3282=CARTESIAN_POINT('',(54.9,-21.8,0.)) ;
#3283=CARTESIAN_POINT('',(54.9,21.6,1.9)) ;
#3284=CARTESIAN_POINT('Origin',(54.9,21.8,1.9)) ;
#3285=CARTESIAN_POINT('',(54.7,21.8,0.)) ;
#3286=CARTESIAN_POINT('',(-54.7,21.8,0.)) ;
#3287=CARTESIAN_POINT('',(54.9,21.8,0.)) ;
#3288=CARTESIAN_POINT('',(-54.7,21.8,1.9)) ;
#3289=CARTESIAN_POINT('',(-54.7,21.8,1.9)) ;
#3290=CARTESIAN_POINT('',(54.7,21.8,1.9)) ;
#3291=CARTESIAN_POINT('',(54.9,21.8,1.9)) ;
#3292=CARTESIAN_POINT('',(54.7,21.8,1.9)) ;
#3293=CARTESIAN_POINT('Origin',(-54.9,-21.8,1.9)) ;
#3294=CARTESIAN_POINT('',(-54.9,-21.6,0.)) ;
#3295=CARTESIAN_POINT('',(-54.9,21.6,0.)) ;
#3296=CARTESIAN_POINT('',(-54.9,-21.8,0.)) ;
#3297=CARTESIAN_POINT('',(-54.9,-21.6,1.9)) ;
#3298=CARTESIAN_POINT('',(-54.9,-21.6,1.9)) ;
#3299=CARTESIAN_POINT('',(-54.9,21.6,1.9)) ;
#3300=CARTESIAN_POINT('',(-54.9,-21.8,1.9)) ;
#3301=CARTESIAN_POINT('',(-54.9,21.6,0.)) ;
#3302=CARTESIAN_POINT('Origin',(54.9,-21.8,1.9)) ;
#3303=CARTESIAN_POINT('',(54.7,-21.8,0.)) ;
#3304=CARTESIAN_POINT('',(-54.7,-21.8,0.)) ;
#3305=CARTESIAN_POINT('',(54.9,-21.8,0.)) ;
#3306=CARTESIAN_POINT('',(54.7,-21.8,1.9)) ;
#3307=CARTESIAN_POINT('',(54.7,-21.8,1.9)) ;
#3308=CARTESIAN_POINT('',(-54.7,-21.8,1.9)) ;
#3309=CARTESIAN_POINT('',(54.9,-21.8,1.9)) ;
#3310=CARTESIAN_POINT('',(-54.7,-21.8,1.9)) ;
#3311=CARTESIAN_POINT('Origin',(0.,0.,1.9)) ;
#3312=CARTESIAN_POINT('Origin',(54.7,-21.6,1.9)) ;
#3313=CARTESIAN_POINT('Origin',(54.7,21.6,1.9)) ;
#3314=CARTESIAN_POINT('Origin',(-54.7,21.6,1.9)) ;
#3315=CARTESIAN_POINT('Origin',(-54.7,-21.6,1.9)) ;
#3316=CARTESIAN_POINT('Origin',(0.,0.,0.)) ;
#3317=CARTESIAN_POINT('Origin',(54.7,-21.6,0.)) ;
#3318=CARTESIAN_POINT('Origin',(-54.7,-21.6,0.)) ;
#3319=CARTESIAN_POINT('Origin',(-54.7,21.6,0.)) ;
#3320=CARTESIAN_POINT('Origin',(54.7,21.6,0.)) ;
#3321=CARTESIAN_POINT('',(23.4,6.00000000000001,0.)) ;
#3322=CARTESIAN_POINT('',(23.4,-6.,0.)) ;
#3323=CARTESIAN_POINT('',(23.4,-6.,0.)) ;
#3324=CARTESIAN_POINT('',(-4.6,6.00000000000001,0.)) ;
#3325=CARTESIAN_POINT('',(-4.6,6.00000000000001,0.)) ;
#3326=CARTESIAN_POINT('',(-4.6,-5.99999999999999,0.)) ;
#3327=CARTESIAN_POINT('',(-4.6,-5.99999999999999,0.)) ;
#3328=CARTESIAN_POINT('',(-4.6,-5.99999999999999,0.)) ;
#3329=CARTESIAN_POINT('',(-45.1,-5.99999999999999,0.)) ;
#3330=CARTESIAN_POINT('',(-45.1,6.00000000000001,0.)) ;
#3331=CARTESIAN_POINT('',(-45.1,-5.99999999999999,0.)) ;
#3332=CARTESIAN_POINT('',(-17.1,-5.99999999999999,0.)) ;
#3333=CARTESIAN_POINT('',(-17.1,-5.99999999999999,0.)) ;
#3334=CARTESIAN_POINT('',(-17.1,6.00000000000001,0.)) ;
#3335=CARTESIAN_POINT('',(-17.1,-5.99999999999999,0.)) ;
#3336=CARTESIAN_POINT('',(-17.1,6.00000000000001,0.)) ;
#3337=CARTESIAN_POINT('Origin',(54.7,-21.6,1.9)) ;
#3338=CARTESIAN_POINT('Origin',(-54.7,-21.6,1.9)) ;
#3339=CARTESIAN_POINT('Origin',(-54.7,21.6,1.9)) ;
#3340=CARTESIAN_POINT('Origin',(54.7,21.6,1.9)) ;
#3341=CARTESIAN_POINT('Origin',(-45.1,-5.99999999999999,6.)) ;
#3342=CARTESIAN_POINT('',(-45.1,-5.99999999999999,6.)) ;
#3343=CARTESIAN_POINT('',(-45.1,6.00000000000001,6.)) ;
#3344=CARTESIAN_POINT('Origin',(-17.1,-5.99999999999999,6.)) ;
#3345=CARTESIAN_POINT('',(-17.1,-5.99999999999999,6.)) ;
#3346=CARTESIAN_POINT('Origin',(-17.1,-5.99999999999999,6.)) ;
#3347=CARTESIAN_POINT('',(-17.1,6.00000000000001,6.)) ;
#3348=CARTESIAN_POINT('Origin',(-17.1,6.00000000000001,6.)) ;
#3349=CARTESIAN_POINT('Origin',(23.4,-6.,6.)) ;
#3350=CARTESIAN_POINT('',(23.4,6.00000000000001,6.)) ;
#3351=CARTESIAN_POINT('',(23.4,-6.,6.)) ;
#3352=CARTESIAN_POINT('Origin',(-4.6,6.00000000000001,6.)) ;
#3353=CARTESIAN_POINT('',(-4.6,6.00000000000001,6.)) ;
#3354=CARTESIAN_POINT('Origin',(-4.6,-5.99999999999999,6.)) ;
#3355=CARTESIAN_POINT('',(-4.6,-5.99999999999999,6.)) ;
#3356=CARTESIAN_POINT('Origin',(-4.6,-5.99999999999999,6.)) ;
#3746=UNCERTAINTY_MEASURE_WITH_UNIT(LENGTH_MEASURE(0.001),#3760,
'DISTANCE_ACCURACY_VALUE',
'Maximum model space distance between geometric entities at asserted c
onnectivities') ;
#3751=UNCERTAINTY_MEASURE_WITH_UNIT(LENGTH_MEASURE(0.001),#3760,
'DISTANCE_ACCURACY_VALUE',
'Maximum model space distance between geometric entities at asserted c
onnectivities') ;
#3754=(
GEOMETRIC_REPRESENTATION_CONTEXT(3)
GLOBAL_UNCERTAINTY_ASSIGNED_CONTEXT((#3746))
GLOBAL_UNIT_ASSIGNED_CONTEXT((#3760,#3762,#3763))
REPRESENTATION_CONTEXT('','3D')
) ;
#3759=(
GEOMETRIC_REPRESENTATION_CONTEXT(3)
GLOBAL_UNCERTAINTY_ASSIGNED_CONTEXT((#3751))
GLOBAL_UNIT_ASSIGNED_CONTEXT((#3760,#3762,#3763))
REPRESENTATION_CONTEXT('','3D')
) ;
#3760=(
LENGTH_UNIT()
NAMED_UNIT(*)
SI_UNIT(.CENTI.,.METRE.)
) ;
#3762=(
NAMED_UNIT(*)
PLANE_ANGLE_UNIT()
SI_UNIT($,.RADIAN.)
) ;
#3763=(
NAMED_UNIT(*)
SI_UNIT($,.STERADIAN.)
SOLID_ANGLE_UNIT()
) ;
#3766=SHAPE_DEFINITION_REPRESENTATION(#3773,#3789) ;
#3773=PRODUCT_DEFINITION_SHAPE('',$,#3797) ;
#3789=SHAPE_REPRESENTATION('',(#2369),#3754) ;
#3794=PRODUCT_DEFINITION_CONTEXT('part definition',#3817,'design') ;
#3797=PRODUCT_DEFINITION('Panel_Top_Side_Inner',
'Panel_Top_Side_Inner',#3804,#3794) ;
#3804=PRODUCT_DEFINITION_FORMATION('',$,#3821) ;
#3817=APPLICATION_CONTEXT(
'Core Data for Automotive Mechanical Design Process') ;
#3818=PRODUCT_CONTEXT('part definition',#3817,'mechanical') ;
#3821=PRODUCT('Panel_Top_Side_Inner','Panel_Top_Side_Inner',$,(#3818)) ;
#3827=PRESENTATION_STYLE_ASSIGNMENT((#3829)) ;
#3829=SURFACE_STYLE_USAGE(.BOTH.,#3831) ;
#3831=SURFACE_SIDE_STYLE('',(#3833)) ;
#3833=SURFACE_STYLE_FILL_AREA(#3835) ;
#3835=FILL_AREA_STYLE('Opaque(179,179,179)',(#3837)) ;
#3837=FILL_AREA_STYLE_COLOUR('Opaque(179,179,179)',#3839) ;
#3839=COLOUR_RGB('Opaque(179,179,179)', 0.09019608, 0.27058824, 0.51372549) ;
ENDSEC;
END-ISO-10303-21;
